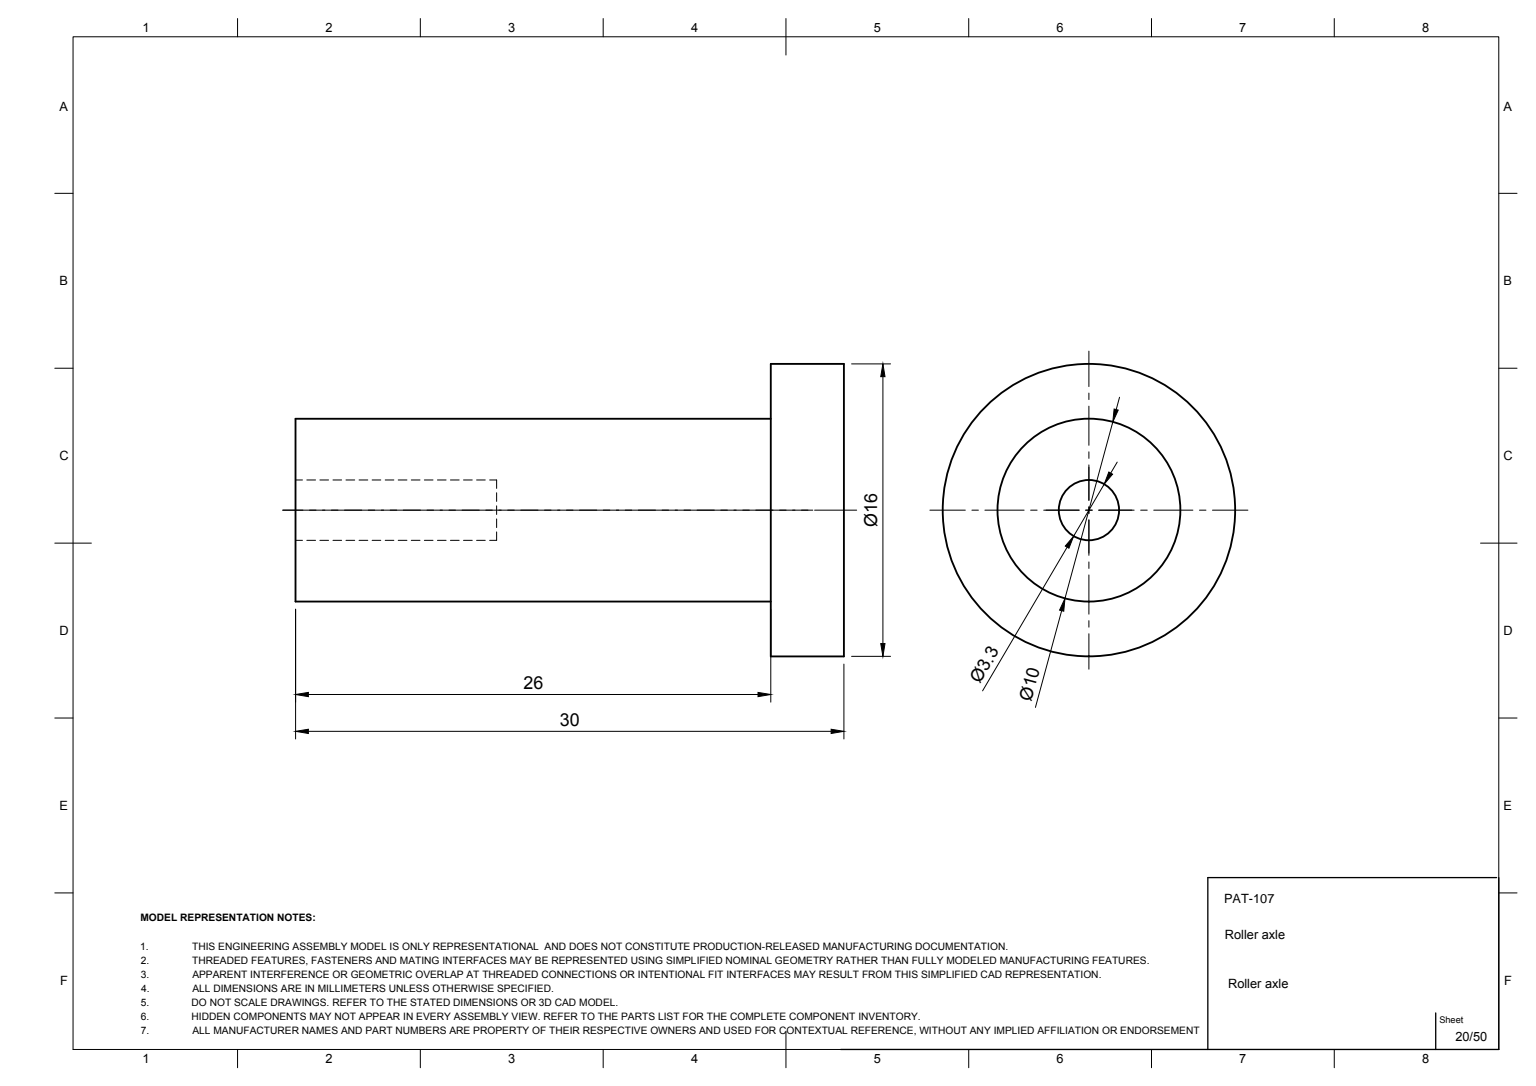
ISO-10303-21;
HEADER;
/* Generated by software containing ST-Developer
 * from STEP Tools, Inc. (www.steptools.com) 
 */

FILE_DESCRIPTION(
/* description */ ('Turntable on roller ring'),
/* implementation_level */ '2;1');

FILE_NAME(
/* name */ 'Roller axle.step',
/* time_stamp */ '2026-10-28T03:23:59-07:00',
/* author */ (''),
/* organization */ (''),
/* preprocessor_version */ 'ST-DEVELOPER v20.2',
/* originating_system */ 'Autodesk Translation Framework v15.17.0.0',
/* authorisation */ '');

FILE_SCHEMA (('AUTOMOTIVE_DESIGN { 1 0 10303 214 3 1 1 }'));
ENDSEC;

DATA;
#10=MECHANICAL_DESIGN_GEOMETRIC_PRESENTATION_REPRESENTATION('',(#643),#16281);
#524=SHAPE_REPRESENTATION_RELATIONSHIP('SRR','None',#16541,#579);
#579=ADVANCED_BREP_SHAPE_REPRESENTATION('',(#713),#16235);
#643=STYLED_ITEM('',(#16932),#713);
#713=MANIFOLD_SOLID_BREP('Body1',#8386);
#881=FACE_BOUND('',#2114,.T.);
#882=FACE_BOUND('',#2119,.T.);
#1099=PLANE('',#9572);
#1100=PLANE('',#9573);
#1101=PLANE('',#9578);
#1102=PLANE('',#9581);
#1482=FACE_OUTER_BOUND('',#2111,.T.);
#1483=FACE_OUTER_BOUND('',#2112,.T.);
#1484=FACE_OUTER_BOUND('',#2113,.T.);
#1485=FACE_OUTER_BOUND('',#2115,.T.);
#1486=FACE_OUTER_BOUND('',#2116,.T.);
#1487=FACE_OUTER_BOUND('',#2117,.T.);
#1488=FACE_OUTER_BOUND('',#2118,.T.);
#2111=EDGE_LOOP('',(#6653,#6654,#6655,#6656));
#2112=EDGE_LOOP('',(#6657));
#2113=EDGE_LOOP('',(#6658));
#2114=EDGE_LOOP('',(#6659));
#2115=EDGE_LOOP('',(#6660,#6661,#6662,#6663));
#2116=EDGE_LOOP('',(#6664));
#2117=EDGE_LOOP('',(#6665,#6666,#6667,#6668));
#2118=EDGE_LOOP('',(#6669));
#2119=EDGE_LOOP('',(#6670));
#2728=LINE('',#14567,#3211);
#2729=LINE('',#14577,#3212);
#2730=LINE('',#14583,#3213);
#3211=VECTOR('',#11497,0.165);
#3212=VECTOR('',#11510,0.8);
#3213=VECTOR('',#11519,0.5);
#3707=CIRCLE('',#9570,0.165);
#3708=CIRCLE('',#9571,0.165);
#3709=CIRCLE('',#9574,0.8);
#3710=CIRCLE('',#9575,0.5);
#3711=CIRCLE('',#9577,0.8);
#3712=CIRCLE('',#9580,0.5);
#4287=VERTEX_POINT('',#14564);
#4288=VERTEX_POINT('',#14566);
#4289=VERTEX_POINT('',#14571);
#4290=VERTEX_POINT('',#14573);
#4291=VERTEX_POINT('',#14576);
#4292=VERTEX_POINT('',#14581);
#5137=EDGE_CURVE('',#4287,#4287,#3707,.T.);
#5138=EDGE_CURVE('',#4287,#4288,#2728,.T.);
#5139=EDGE_CURVE('',#4288,#4288,#3708,.T.);
#5140=EDGE_CURVE('',#4289,#4289,#3709,.T.);
#5141=EDGE_CURVE('',#4290,#4290,#3710,.T.);
#5142=EDGE_CURVE('',#4289,#4291,#2729,.T.);
#5143=EDGE_CURVE('',#4291,#4291,#3711,.T.);
#5144=EDGE_CURVE('',#4292,#4292,#3712,.T.);
#5145=EDGE_CURVE('',#4292,#4290,#2730,.T.);
#6653=ORIENTED_EDGE('',*,*,#5137,.F.);
#6654=ORIENTED_EDGE('',*,*,#5138,.T.);
#6655=ORIENTED_EDGE('',*,*,#5139,.F.);
#6656=ORIENTED_EDGE('',*,*,#5138,.F.);
#6657=ORIENTED_EDGE('',*,*,#5137,.T.);
#6658=ORIENTED_EDGE('',*,*,#5140,.T.);
#6659=ORIENTED_EDGE('',*,*,#5141,.F.);
#6660=ORIENTED_EDGE('',*,*,#5140,.F.);
#6661=ORIENTED_EDGE('',*,*,#5142,.T.);
#6662=ORIENTED_EDGE('',*,*,#5143,.T.);
#6663=ORIENTED_EDGE('',*,*,#5142,.F.);
#6664=ORIENTED_EDGE('',*,*,#5143,.F.);
#6665=ORIENTED_EDGE('',*,*,#5144,.F.);
#6666=ORIENTED_EDGE('',*,*,#5145,.T.);
#6667=ORIENTED_EDGE('',*,*,#5141,.T.);
#6668=ORIENTED_EDGE('',*,*,#5145,.F.);
#6669=ORIENTED_EDGE('',*,*,#5144,.T.);
#6670=ORIENTED_EDGE('',*,*,#5139,.T.);
#7759=CYLINDRICAL_SURFACE('',#9569,0.165);
#7760=CYLINDRICAL_SURFACE('',#9576,0.8);
#7761=CYLINDRICAL_SURFACE('',#9579,0.5);
#8085=ADVANCED_FACE('',(#1482),#7759,.F.);
#8086=ADVANCED_FACE('',(#1483),#1099,.T.);
#8087=ADVANCED_FACE('',(#1484,#881),#1100,.T.);
#8088=ADVANCED_FACE('',(#1485),#7760,.T.);
#8089=ADVANCED_FACE('',(#1486),#1101,.F.);
#8090=ADVANCED_FACE('',(#1487),#7761,.T.);
#8091=ADVANCED_FACE('',(#1488,#882),#1102,.T.);
#8386=CLOSED_SHELL('',(#8085,#8086,#8087,#8088,#8089,#8090,#8091));
#9568=AXIS2_PLACEMENT_3D('',#14562,#11491,#11492);
#9569=AXIS2_PLACEMENT_3D('',#14563,#11493,#11494);
#9570=AXIS2_PLACEMENT_3D('',#14565,#11495,#11496);
#9571=AXIS2_PLACEMENT_3D('',#14568,#11498,#11499);
#9572=AXIS2_PLACEMENT_3D('',#14569,#11500,#11501);
#9573=AXIS2_PLACEMENT_3D('',#14570,#11502,#11503);
#9574=AXIS2_PLACEMENT_3D('',#14572,#11504,#11505);
#9575=AXIS2_PLACEMENT_3D('',#14574,#11506,#11507);
#9576=AXIS2_PLACEMENT_3D('',#14575,#11508,#11509);
#9577=AXIS2_PLACEMENT_3D('',#14578,#11511,#11512);
#9578=AXIS2_PLACEMENT_3D('',#14579,#11513,#11514);
#9579=AXIS2_PLACEMENT_3D('',#14580,#11515,#11516);
#9580=AXIS2_PLACEMENT_3D('',#14582,#11517,#11518);
#9581=AXIS2_PLACEMENT_3D('',#14584,#11520,#11521);
#11491=DIRECTION('axis',(0.,0.,1.));
#11492=DIRECTION('refdir',(1.,0.,0.));
#11493=DIRECTION('center_axis',(0.,1.,0.));
#11494=DIRECTION('ref_axis',(1.,0.,0.));
#11495=DIRECTION('center_axis',(0.,1.,0.));
#11496=DIRECTION('ref_axis',(1.,0.,0.));
#11497=DIRECTION('',(0.,1.,0.));
#11498=DIRECTION('center_axis',(0.,-1.,0.));
#11499=DIRECTION('ref_axis',(1.,0.,0.));
#11500=DIRECTION('center_axis',(0.,1.,0.));
#11501=DIRECTION('ref_axis',(1.,0.,0.));
#11502=DIRECTION('center_axis',(0.,1.,0.));
#11503=DIRECTION('ref_axis',(1.,0.,0.));
#11504=DIRECTION('center_axis',(0.,1.,0.));
#11505=DIRECTION('ref_axis',(1.,0.,0.));
#11506=DIRECTION('center_axis',(0.,1.,0.));
#11507=DIRECTION('ref_axis',(1.,0.,0.));
#11508=DIRECTION('center_axis',(0.,1.,0.));
#11509=DIRECTION('ref_axis',(1.,0.,0.));
#11510=DIRECTION('',(0.,-1.,0.));
#11511=DIRECTION('center_axis',(0.,1.,0.));
#11512=DIRECTION('ref_axis',(1.,0.,0.));
#11513=DIRECTION('center_axis',(0.,1.,0.));
#11514=DIRECTION('ref_axis',(1.,0.,0.));
#11515=DIRECTION('center_axis',(0.,1.,0.));
#11516=DIRECTION('ref_axis',(1.,0.,0.));
#11517=DIRECTION('center_axis',(0.,1.,0.));
#11518=DIRECTION('ref_axis',(1.,0.,0.));
#11519=DIRECTION('',(0.,-1.,0.));
#11520=DIRECTION('center_axis',(0.,1.,0.));
#11521=DIRECTION('ref_axis',(1.,0.,0.));
#14562=CARTESIAN_POINT('',(0.,0.,0.));
#14563=CARTESIAN_POINT('Origin',(0.,15.2,3.5));
#14564=CARTESIAN_POINT('',(-0.165,15.2,3.5));
#14565=CARTESIAN_POINT('Origin',(0.,15.2,3.5));
#14566=CARTESIAN_POINT('',(-0.165,16.3,3.5));
#14567=CARTESIAN_POINT('',(-0.165,15.2,3.5));
#14568=CARTESIAN_POINT('Origin',(0.,16.3,3.5));
#14569=CARTESIAN_POINT('Origin',(0.,15.2,3.5));
#14570=CARTESIAN_POINT('Origin',(0.,13.7,3.5));
#14571=CARTESIAN_POINT('',(-0.8,13.7,3.5));
#14572=CARTESIAN_POINT('Origin',(0.,13.7,3.5));
#14573=CARTESIAN_POINT('',(-0.5,13.7,3.5));
#14574=CARTESIAN_POINT('Origin',(0.,13.7,3.5));
#14575=CARTESIAN_POINT('Origin',(0.,13.3,3.5));
#14576=CARTESIAN_POINT('',(-0.8,13.3,3.5));
#14577=CARTESIAN_POINT('',(-0.8,13.3,3.5));
#14578=CARTESIAN_POINT('Origin',(0.,13.3,3.5));
#14579=CARTESIAN_POINT('Origin',(0.,13.3,3.5));
#14580=CARTESIAN_POINT('Origin',(0.,13.7,3.5));
#14581=CARTESIAN_POINT('',(-0.5,16.3,3.5));
#14582=CARTESIAN_POINT('Origin',(0.,16.3,3.5));
#14583=CARTESIAN_POINT('',(-0.5,13.7,3.5));
#14584=CARTESIAN_POINT('Origin',(0.,16.3,3.5));
#16166=UNCERTAINTY_MEASURE_WITH_UNIT(LENGTH_MEASURE(0.001),#16282,
'DISTANCE_ACCURACY_VALUE',
'Maximum model space distance between geometric entities at asserted c
onnectivities');
#16212=UNCERTAINTY_MEASURE_WITH_UNIT(LENGTH_MEASURE(0.001),#16282,
'DISTANCE_ACCURACY_VALUE',
'Maximum model space distance between geometric entities at asserted c
onnectivities');
#16235=(
GEOMETRIC_REPRESENTATION_CONTEXT(3)
GLOBAL_UNCERTAINTY_ASSIGNED_CONTEXT((#16166))
GLOBAL_UNIT_ASSIGNED_CONTEXT((#16282,#16284,#16285))
REPRESENTATION_CONTEXT('','3D')
);
#16281=(
GEOMETRIC_REPRESENTATION_CONTEXT(3)
GLOBAL_UNCERTAINTY_ASSIGNED_CONTEXT((#16212))
GLOBAL_UNIT_ASSIGNED_CONTEXT((#16282,#16284,#16285))
REPRESENTATION_CONTEXT('','3D')
);
#16282=(
LENGTH_UNIT()
NAMED_UNIT(*)
SI_UNIT(.CENTI.,.METRE.)
);
#16284=(
NAMED_UNIT(*)
PLANE_ANGLE_UNIT()
SI_UNIT($,.RADIAN.)
);
#16285=(
NAMED_UNIT(*)
SI_UNIT($,.STERADIAN.)
SOLID_ANGLE_UNIT()
);
#16308=SHAPE_DEFINITION_REPRESENTATION(#16402,#16541);
#16402=PRODUCT_DEFINITION_SHAPE('',$,#16610);
#16541=SHAPE_REPRESENTATION('',(#9568),#16235);
#16587=PRODUCT_DEFINITION_CONTEXT('part definition',#16793,'design');
#16610=PRODUCT_DEFINITION('Roller axle','Roller axle',#16678,#16587);
#16678=PRODUCT_DEFINITION_FORMATION('',$,#16817);
#16793=APPLICATION_CONTEXT(
'Core Data for Automotive Mechanical Design Process');
#16794=PRODUCT_CONTEXT('part definition',#16793,'mechanical');
#16817=PRODUCT('Roller axle','Roller axle','Roller axle',(#16794));
#16926=COLOUR_RGB('Grey',0.48,0.52,0.57);
#16927=FILL_AREA_STYLE_COLOUR('',#16926);
#16928=FILL_AREA_STYLE('',(#16927));
#16929=SURFACE_STYLE_FILL_AREA(#16928);
#16930=SURFACE_SIDE_STYLE('',(#16929));
#16931=SURFACE_STYLE_USAGE(.BOTH.,#16930);
#16932=PRESENTATION_STYLE_ASSIGNMENT((#16931));
ENDSEC;
END-ISO-10303-21;
